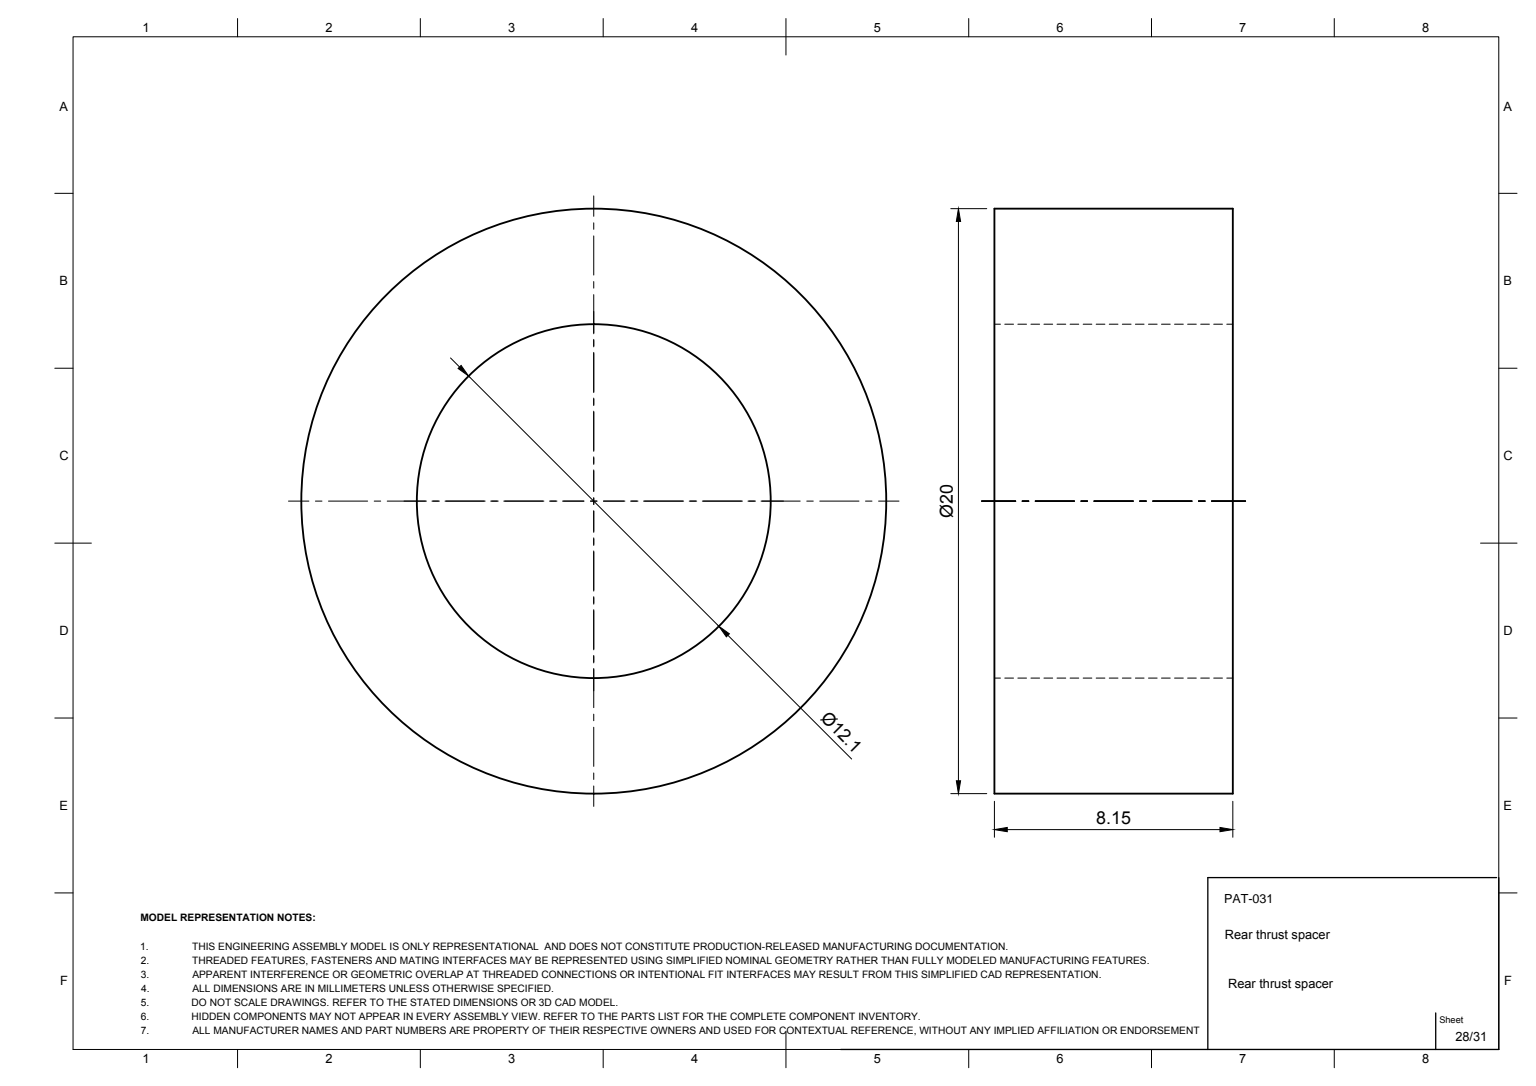
ISO-10303-21;
HEADER;
/* Generated by software containing ST-Developer
 * from STEP Tools, Inc. (www.steptools.com) 
 */

FILE_DESCRIPTION(
/* description */ ('Double-row support with tensioned shaft'),
/* implementation_level */ '2;1');

FILE_NAME(
/* name */ 'Rear thrust spacer.step',
/* time_stamp */ '2026-10-27T10:50:35-07:00',
/* author */ (''),
/* organization */ (''),
/* preprocessor_version */ 'ST-DEVELOPER v20.2',
/* originating_system */ 'Autodesk Translation Framework v15.17.0.0',
/* authorisation */ '');

FILE_SCHEMA (('AUTOMOTIVE_DESIGN { 1 0 10303 214 3 1 1 }'));
ENDSEC;

DATA;
#10=MECHANICAL_DESIGN_GEOMETRIC_PRESENTATION_REPRESENTATION('',(#505),#11559);
#440=SHAPE_REPRESENTATION_RELATIONSHIP('SRR','None',#11750,#472);
#472=ADVANCED_BREP_SHAPE_REPRESENTATION('',(#535),#11552);
#505=STYLED_ITEM('',(#11953),#535);
#535=MANIFOLD_SOLID_BREP('Body1',#6353);
#656=FACE_BOUND('',#1656,.T.);
#657=FACE_BOUND('',#1658,.T.);
#869=PLANE('',#7260);
#870=PLANE('',#7261);
#1195=FACE_OUTER_BOUND('',#1653,.T.);
#1196=FACE_OUTER_BOUND('',#1654,.T.);
#1197=FACE_OUTER_BOUND('',#1655,.T.);
#1198=FACE_OUTER_BOUND('',#1657,.T.);
#1653=EDGE_LOOP('',(#5598,#5599,#5600,#5601));
#1654=EDGE_LOOP('',(#5602,#5603,#5604,#5605));
#1655=EDGE_LOOP('',(#5606));
#1656=EDGE_LOOP('',(#5607));
#1657=EDGE_LOOP('',(#5608));
#1658=EDGE_LOOP('',(#5609));
#2182=LINE('',#11113,#2729);
#2183=LINE('',#11119,#2730);
#2729=VECTOR('',#8897,0.605);
#2730=VECTOR('',#8904,1.);
#2992=CIRCLE('',#7255,0.605);
#2993=CIRCLE('',#7256,0.605);
#2994=CIRCLE('',#7258,1.);
#2995=CIRCLE('',#7259,1.);
#3453=VERTEX_POINT('',#11110);
#3454=VERTEX_POINT('',#11112);
#3455=VERTEX_POINT('',#11116);
#3456=VERTEX_POINT('',#11118);
#4184=EDGE_CURVE('',#3453,#3453,#2992,.T.);
#4185=EDGE_CURVE('',#3453,#3454,#2182,.T.);
#4186=EDGE_CURVE('',#3454,#3454,#2993,.T.);
#4187=EDGE_CURVE('',#3455,#3455,#2994,.T.);
#4188=EDGE_CURVE('',#3455,#3456,#2183,.T.);
#4189=EDGE_CURVE('',#3456,#3456,#2995,.T.);
#5598=ORIENTED_EDGE('',*,*,#4184,.F.);
#5599=ORIENTED_EDGE('',*,*,#4185,.T.);
#5600=ORIENTED_EDGE('',*,*,#4186,.T.);
#5601=ORIENTED_EDGE('',*,*,#4185,.F.);
#5602=ORIENTED_EDGE('',*,*,#4187,.F.);
#5603=ORIENTED_EDGE('',*,*,#4188,.T.);
#5604=ORIENTED_EDGE('',*,*,#4189,.T.);
#5605=ORIENTED_EDGE('',*,*,#4188,.F.);
#5606=ORIENTED_EDGE('',*,*,#4187,.T.);
#5607=ORIENTED_EDGE('',*,*,#4184,.T.);
#5608=ORIENTED_EDGE('',*,*,#4189,.F.);
#5609=ORIENTED_EDGE('',*,*,#4186,.F.);
#5964=CYLINDRICAL_SURFACE('',#7254,0.605);
#5965=CYLINDRICAL_SURFACE('',#7257,1.);
#6258=ADVANCED_FACE('',(#1195),#5964,.F.);
#6259=ADVANCED_FACE('',(#1196),#5965,.T.);
#6260=ADVANCED_FACE('',(#1197,#656),#869,.T.);
#6261=ADVANCED_FACE('',(#1198,#657),#870,.F.);
#6353=CLOSED_SHELL('',(#6258,#6259,#6260,#6261));
#7253=AXIS2_PLACEMENT_3D('',#11108,#8891,#8892);
#7254=AXIS2_PLACEMENT_3D('',#11109,#8893,#8894);
#7255=AXIS2_PLACEMENT_3D('',#11111,#8895,#8896);
#7256=AXIS2_PLACEMENT_3D('',#11114,#8898,#8899);
#7257=AXIS2_PLACEMENT_3D('',#11115,#8900,#8901);
#7258=AXIS2_PLACEMENT_3D('',#11117,#8902,#8903);
#7259=AXIS2_PLACEMENT_3D('',#11120,#8905,#8906);
#7260=AXIS2_PLACEMENT_3D('',#11121,#8907,#8908);
#7261=AXIS2_PLACEMENT_3D('',#11122,#8909,#8910);
#8891=DIRECTION('axis',(0.,0.,1.));
#8892=DIRECTION('refdir',(1.,0.,0.));
#8893=DIRECTION('center_axis',(0.,1.,0.));
#8894=DIRECTION('ref_axis',(1.,0.,0.));
#8895=DIRECTION('center_axis',(0.,-1.,0.));
#8896=DIRECTION('ref_axis',(1.,0.,0.));
#8897=DIRECTION('',(0.,-1.,0.));
#8898=DIRECTION('center_axis',(0.,-1.,0.));
#8899=DIRECTION('ref_axis',(1.,0.,0.));
#8900=DIRECTION('center_axis',(0.,1.,0.));
#8901=DIRECTION('ref_axis',(1.,0.,0.));
#8902=DIRECTION('center_axis',(0.,1.,0.));
#8903=DIRECTION('ref_axis',(1.,0.,0.));
#8904=DIRECTION('',(0.,-1.,0.));
#8905=DIRECTION('center_axis',(0.,1.,0.));
#8906=DIRECTION('ref_axis',(1.,0.,0.));
#8907=DIRECTION('center_axis',(0.,1.,0.));
#8908=DIRECTION('ref_axis',(1.,0.,0.));
#8909=DIRECTION('center_axis',(0.,1.,0.));
#8910=DIRECTION('ref_axis',(1.,0.,0.));
#11108=CARTESIAN_POINT('',(0.,0.,0.));
#11109=CARTESIAN_POINT('Origin',(0.,-1.665,10.));
#11110=CARTESIAN_POINT('',(-0.605,-0.85,10.));
#11111=CARTESIAN_POINT('Origin',(0.,-0.85,10.));
#11112=CARTESIAN_POINT('',(-0.605,-1.665,10.));
#11113=CARTESIAN_POINT('',(-0.605,-1.665,10.));
#11114=CARTESIAN_POINT('Origin',(0.,-1.665,10.));
#11115=CARTESIAN_POINT('Origin',(0.,-1.665,10.));
#11116=CARTESIAN_POINT('',(-1.,-0.85,10.));
#11117=CARTESIAN_POINT('Origin',(0.,-0.85,10.));
#11118=CARTESIAN_POINT('',(-1.,-1.665,10.));
#11119=CARTESIAN_POINT('',(-1.,-1.665,10.));
#11120=CARTESIAN_POINT('Origin',(0.,-1.665,10.));
#11121=CARTESIAN_POINT('Origin',(0.,-0.85,10.));
#11122=CARTESIAN_POINT('Origin',(0.,-1.665,10.));
#11515=UNCERTAINTY_MEASURE_WITH_UNIT(LENGTH_MEASURE(0.001),#11560,
'DISTANCE_ACCURACY_VALUE',
'Maximum model space distance between geometric entities at asserted c
onnectivities');
#11522=UNCERTAINTY_MEASURE_WITH_UNIT(LENGTH_MEASURE(0.001),#11560,
'DISTANCE_ACCURACY_VALUE',
'Maximum model space distance between geometric entities at asserted c
onnectivities');
#11552=(
GEOMETRIC_REPRESENTATION_CONTEXT(3)
GLOBAL_UNCERTAINTY_ASSIGNED_CONTEXT((#11515))
GLOBAL_UNIT_ASSIGNED_CONTEXT((#11560,#11562,#11563))
REPRESENTATION_CONTEXT('','3D')
);
#11559=(
GEOMETRIC_REPRESENTATION_CONTEXT(3)
GLOBAL_UNCERTAINTY_ASSIGNED_CONTEXT((#11522))
GLOBAL_UNIT_ASSIGNED_CONTEXT((#11560,#11562,#11563))
REPRESENTATION_CONTEXT('','3D')
);
#11560=(
LENGTH_UNIT()
NAMED_UNIT(*)
SI_UNIT(.CENTI.,.METRE.)
);
#11562=(
NAMED_UNIT(*)
PLANE_ANGLE_UNIT()
SI_UNIT($,.RADIAN.)
);
#11563=(
NAMED_UNIT(*)
SI_UNIT($,.STERADIAN.)
SOLID_ANGLE_UNIT()
);
#11593=SHAPE_DEFINITION_REPRESENTATION(#11704,#11750);
#11704=PRODUCT_DEFINITION_SHAPE('',$,#11787);
#11750=SHAPE_REPRESENTATION('',(#7253),#11552);
#11757=PRODUCT_DEFINITION_CONTEXT('part definition',#11867,'design');
#11787=PRODUCT_DEFINITION('Rear thrust spacer','Rear thrust spacer',#11823,
#11757);
#11823=PRODUCT_DEFINITION_FORMATION('',$,#11898);
#11867=APPLICATION_CONTEXT(
'Core Data for Automotive Mechanical Design Process');
#11868=PRODUCT_CONTEXT('part definition',#11867,'mechanical');
#11898=PRODUCT('Rear thrust spacer','Rear thrust spacer',
'Rear thrust spacer',(#11868));
#11947=COLOUR_RGB('Light Blue',0.38,0.62,0.78);
#11948=FILL_AREA_STYLE_COLOUR('',#11947);
#11949=FILL_AREA_STYLE('',(#11948));
#11950=SURFACE_STYLE_FILL_AREA(#11949);
#11951=SURFACE_SIDE_STYLE('',(#11950));
#11952=SURFACE_STYLE_USAGE(.BOTH.,#11951);
#11953=PRESENTATION_STYLE_ASSIGNMENT((#11952));
ENDSEC;
END-ISO-10303-21;
